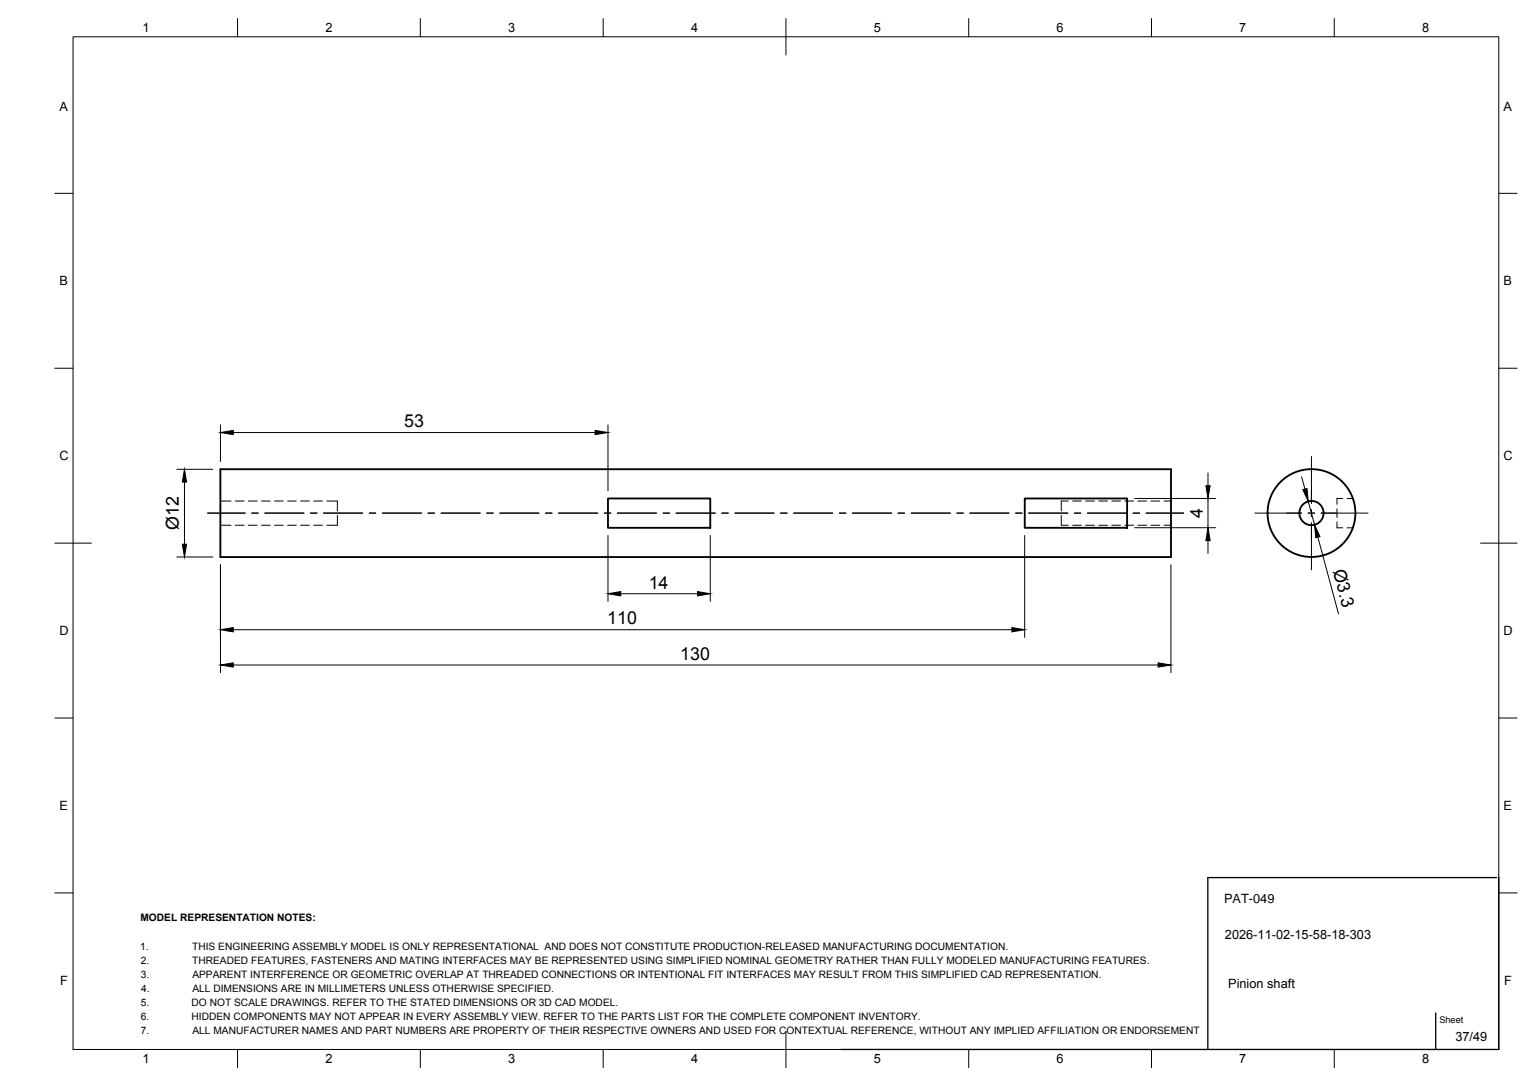
ISO-10303-21;
HEADER;
/* Generated by software containing ST-Developer
 * from STEP Tools, Inc. (www.steptools.com) 
 */

FILE_DESCRIPTION(
/* description */ ('Hand drill press frame (manual)'),
/* implementation_level */ '2;1');

FILE_NAME(
/* name */ 'Pinion shaft.step',
/* time_stamp */ '2026-10-28T03:25:28-07:00',
/* author */ (''),
/* organization */ (''),
/* preprocessor_version */ 'ST-DEVELOPER v20.2',
/* originating_system */ 'Autodesk Translation Framework v15.17.0.0',
/* authorisation */ '');

FILE_SCHEMA (('AUTOMOTIVE_DESIGN { 1 0 10303 214 3 1 1 }'));
ENDSEC;

DATA;
#10=MECHANICAL_DESIGN_GEOMETRIC_PRESENTATION_REPRESENTATION('',(#655),#33299);
#558=SHAPE_REPRESENTATION_RELATIONSHIP('SRR','None',#33520,#603);
#603=ADVANCED_BREP_SHAPE_REPRESENTATION('',(#706),#33282);
#655=STYLED_ITEM('',(#33814),#706);
#706=MANIFOLD_SOLID_BREP('Body1',#12674);
#855=FACE_BOUND('',#2667,.T.);
#856=FACE_BOUND('',#2668,.T.);
#857=FACE_BOUND('',#2670,.T.);
#858=FACE_BOUND('',#2672,.T.);
#1238=PLANE('',#14009);
#1239=PLANE('',#14013);
#1240=PLANE('',#14014);
#1241=PLANE('',#14015);
#1242=PLANE('',#14017);
#1243=PLANE('',#14018);
#1244=PLANE('',#14019);
#1245=PLANE('',#14021);
#1246=PLANE('',#14022);
#1247=PLANE('',#14024);
#1248=PLANE('',#14025);
#1249=PLANE('',#14026);
#1250=PLANE('',#14031);
#1251=PLANE('',#14032);
#1828=FACE_OUTER_BOUND('',#2652,.T.);
#1829=FACE_OUTER_BOUND('',#2653,.T.);
#1830=FACE_OUTER_BOUND('',#2654,.T.);
#1831=FACE_OUTER_BOUND('',#2655,.T.);
#1832=FACE_OUTER_BOUND('',#2656,.T.);
#1833=FACE_OUTER_BOUND('',#2657,.T.);
#1834=FACE_OUTER_BOUND('',#2658,.T.);
#1835=FACE_OUTER_BOUND('',#2659,.T.);
#1836=FACE_OUTER_BOUND('',#2660,.T.);
#1837=FACE_OUTER_BOUND('',#2661,.T.);
#1838=FACE_OUTER_BOUND('',#2662,.T.);
#1839=FACE_OUTER_BOUND('',#2663,.T.);
#1840=FACE_OUTER_BOUND('',#2664,.T.);
#1841=FACE_OUTER_BOUND('',#2665,.T.);
#1842=FACE_OUTER_BOUND('',#2666,.T.);
#1843=FACE_OUTER_BOUND('',#2669,.T.);
#1844=FACE_OUTER_BOUND('',#2671,.T.);
#2652=EDGE_LOOP('',(#10865,#10866,#10867,#10868));
#2653=EDGE_LOOP('',(#10869));
#2654=EDGE_LOOP('',(#10870,#10871,#10872,#10873));
#2655=EDGE_LOOP('',(#10874));
#2656=EDGE_LOOP('',(#10875,#10876,#10877,#10878));
#2657=EDGE_LOOP('',(#10879,#10880,#10881,#10882));
#2658=EDGE_LOOP('',(#10883,#10884,#10885,#10886));
#2659=EDGE_LOOP('',(#10887,#10888,#10889,#10890));
#2660=EDGE_LOOP('',(#10891,#10892,#10893,#10894));
#2661=EDGE_LOOP('',(#10895,#10896,#10897,#10898));
#2662=EDGE_LOOP('',(#10899,#10900,#10901,#10902));
#2663=EDGE_LOOP('',(#10903,#10904,#10905,#10906));
#2664=EDGE_LOOP('',(#10907,#10908,#10909,#10910));
#2665=EDGE_LOOP('',(#10911,#10912,#10913,#10914));
#2666=EDGE_LOOP('',(#10915,#10916,#10917,#10918));
#2667=EDGE_LOOP('',(#10919,#10920,#10921,#10922));
#2668=EDGE_LOOP('',(#10923,#10924,#10925,#10926));
#2669=EDGE_LOOP('',(#10927));
#2670=EDGE_LOOP('',(#10928));
#2671=EDGE_LOOP('',(#10929));
#2672=EDGE_LOOP('',(#10930));
#3785=LINE('',#21071,#4950);
#3786=LINE('',#21078,#4951);
#3787=LINE('',#21084,#4952);
#3788=LINE('',#21086,#4953);
#3789=LINE('',#21088,#4954);
#3790=LINE('',#21089,#4955);
#3791=LINE('',#21094,#4956);
#3792=LINE('',#21095,#4957);
#3793=LINE('',#21098,#4958);
#3794=LINE('',#21099,#4959);
#3795=LINE('',#21102,#4960);
#3796=LINE('',#21103,#4961);
#3797=LINE('',#21109,#4962);
#3798=LINE('',#21111,#4963);
#3799=LINE('',#21113,#4964);
#3800=LINE('',#21114,#4965);
#3801=LINE('',#21119,#4966);
#3802=LINE('',#21120,#4967);
#3803=LINE('',#21123,#4968);
#3804=LINE('',#21124,#4969);
#3805=LINE('',#21127,#4970);
#3806=LINE('',#21128,#4971);
#3807=LINE('',#21135,#4972);
#4950=VECTOR('',#16908,0.165);
#4951=VECTOR('',#16917,0.165);
#4952=VECTOR('',#16924,1.);
#4953=VECTOR('',#16925,1.);
#4954=VECTOR('',#16926,1.);
#4955=VECTOR('',#16927,1.);
#4956=VECTOR('',#16932,1.);
#4957=VECTOR('',#16933,1.);
#4958=VECTOR('',#16936,1.);
#4959=VECTOR('',#16937,1.);
#4960=VECTOR('',#16940,1.);
#4961=VECTOR('',#16941,1.);
#4962=VECTOR('',#16948,1.);
#4963=VECTOR('',#16949,1.);
#4964=VECTOR('',#16950,1.);
#4965=VECTOR('',#16951,1.);
#4966=VECTOR('',#16956,1.);
#4967=VECTOR('',#16957,1.);
#4968=VECTOR('',#16960,1.);
#4969=VECTOR('',#16961,1.);
#4970=VECTOR('',#16964,1.);
#4971=VECTOR('',#16965,1.);
#4972=VECTOR('',#16974,0.6);
#5497=CIRCLE('',#14007,0.165);
#5498=CIRCLE('',#14008,0.165);
#5499=CIRCLE('',#14011,0.165);
#5500=CIRCLE('',#14012,0.165);
#5501=CIRCLE('',#14016,0.6);
#5502=CIRCLE('',#14020,0.6);
#5503=CIRCLE('',#14023,0.6);
#5504=CIRCLE('',#14027,0.6);
#5505=CIRCLE('',#14029,0.6);
#5506=CIRCLE('',#14030,0.6);
#6435=VERTEX_POINT('',#21068);
#6436=VERTEX_POINT('',#21070);
#6437=VERTEX_POINT('',#21075);
#6438=VERTEX_POINT('',#21077);
#6439=VERTEX_POINT('',#21082);
#6440=VERTEX_POINT('',#21083);
#6441=VERTEX_POINT('',#21085);
#6442=VERTEX_POINT('',#21087);
#6443=VERTEX_POINT('',#21091);
#6444=VERTEX_POINT('',#21093);
#6445=VERTEX_POINT('',#21097);
#6446=VERTEX_POINT('',#21101);
#6447=VERTEX_POINT('',#21107);
#6448=VERTEX_POINT('',#21108);
#6449=VERTEX_POINT('',#21110);
#6450=VERTEX_POINT('',#21112);
#6451=VERTEX_POINT('',#21116);
#6452=VERTEX_POINT('',#21118);
#6453=VERTEX_POINT('',#21122);
#6454=VERTEX_POINT('',#21126);
#6455=VERTEX_POINT('',#21132);
#6456=VERTEX_POINT('',#21134);
#7961=EDGE_CURVE('',#6435,#6435,#5497,.T.);
#7962=EDGE_CURVE('',#6435,#6436,#3785,.T.);
#7963=EDGE_CURVE('',#6436,#6436,#5498,.T.);
#7964=EDGE_CURVE('',#6437,#6437,#5499,.T.);
#7965=EDGE_CURVE('',#6437,#6438,#3786,.T.);
#7966=EDGE_CURVE('',#6438,#6438,#5500,.T.);
#7967=EDGE_CURVE('',#6439,#6440,#3787,.T.);
#7968=EDGE_CURVE('',#6439,#6441,#3788,.T.);
#7969=EDGE_CURVE('',#6442,#6441,#3789,.T.);
#7970=EDGE_CURVE('',#6442,#6440,#3790,.T.);
#7971=EDGE_CURVE('',#6440,#6443,#5501,.T.);
#7972=EDGE_CURVE('',#6444,#6442,#3791,.T.);
#7973=EDGE_CURVE('',#6443,#6444,#3792,.T.);
#7974=EDGE_CURVE('',#6441,#6445,#3793,.T.);
#7975=EDGE_CURVE('',#6444,#6445,#3794,.T.);
#7976=EDGE_CURVE('',#6443,#6446,#3795,.T.);
#7977=EDGE_CURVE('',#6445,#6446,#3796,.T.);
#7978=EDGE_CURVE('',#6446,#6439,#5502,.T.);
#7979=EDGE_CURVE('',#6447,#6448,#3797,.T.);
#7980=EDGE_CURVE('',#6447,#6449,#3798,.T.);
#7981=EDGE_CURVE('',#6450,#6449,#3799,.T.);
#7982=EDGE_CURVE('',#6450,#6448,#3800,.T.);
#7983=EDGE_CURVE('',#6448,#6451,#5503,.T.);
#7984=EDGE_CURVE('',#6452,#6450,#3801,.T.);
#7985=EDGE_CURVE('',#6451,#6452,#3802,.T.);
#7986=EDGE_CURVE('',#6449,#6453,#3803,.T.);
#7987=EDGE_CURVE('',#6452,#6453,#3804,.T.);
#7988=EDGE_CURVE('',#6451,#6454,#3805,.T.);
#7989=EDGE_CURVE('',#6453,#6454,#3806,.T.);
#7990=EDGE_CURVE('',#6454,#6447,#5504,.T.);
#7991=EDGE_CURVE('',#6455,#6455,#5505,.T.);
#7992=EDGE_CURVE('',#6455,#6456,#3807,.T.);
#7993=EDGE_CURVE('',#6456,#6456,#5506,.T.);
#10865=ORIENTED_EDGE('',*,*,#7961,.F.);
#10866=ORIENTED_EDGE('',*,*,#7962,.T.);
#10867=ORIENTED_EDGE('',*,*,#7963,.F.);
#10868=ORIENTED_EDGE('',*,*,#7962,.F.);
#10869=ORIENTED_EDGE('',*,*,#7961,.T.);
#10870=ORIENTED_EDGE('',*,*,#7964,.F.);
#10871=ORIENTED_EDGE('',*,*,#7965,.T.);
#10872=ORIENTED_EDGE('',*,*,#7966,.T.);
#10873=ORIENTED_EDGE('',*,*,#7965,.F.);
#10874=ORIENTED_EDGE('',*,*,#7966,.F.);
#10875=ORIENTED_EDGE('',*,*,#7967,.F.);
#10876=ORIENTED_EDGE('',*,*,#7968,.T.);
#10877=ORIENTED_EDGE('',*,*,#7969,.F.);
#10878=ORIENTED_EDGE('',*,*,#7970,.T.);
#10879=ORIENTED_EDGE('',*,*,#7971,.F.);
#10880=ORIENTED_EDGE('',*,*,#7970,.F.);
#10881=ORIENTED_EDGE('',*,*,#7972,.F.);
#10882=ORIENTED_EDGE('',*,*,#7973,.F.);
#10883=ORIENTED_EDGE('',*,*,#7972,.T.);
#10884=ORIENTED_EDGE('',*,*,#7969,.T.);
#10885=ORIENTED_EDGE('',*,*,#7974,.T.);
#10886=ORIENTED_EDGE('',*,*,#7975,.F.);
#10887=ORIENTED_EDGE('',*,*,#7976,.F.);
#10888=ORIENTED_EDGE('',*,*,#7973,.T.);
#10889=ORIENTED_EDGE('',*,*,#7975,.T.);
#10890=ORIENTED_EDGE('',*,*,#7977,.T.);
#10891=ORIENTED_EDGE('',*,*,#7978,.F.);
#10892=ORIENTED_EDGE('',*,*,#7977,.F.);
#10893=ORIENTED_EDGE('',*,*,#7974,.F.);
#10894=ORIENTED_EDGE('',*,*,#7968,.F.);
#10895=ORIENTED_EDGE('',*,*,#7979,.F.);
#10896=ORIENTED_EDGE('',*,*,#7980,.T.);
#10897=ORIENTED_EDGE('',*,*,#7981,.F.);
#10898=ORIENTED_EDGE('',*,*,#7982,.T.);
#10899=ORIENTED_EDGE('',*,*,#7983,.F.);
#10900=ORIENTED_EDGE('',*,*,#7982,.F.);
#10901=ORIENTED_EDGE('',*,*,#7984,.F.);
#10902=ORIENTED_EDGE('',*,*,#7985,.F.);
#10903=ORIENTED_EDGE('',*,*,#7984,.T.);
#10904=ORIENTED_EDGE('',*,*,#7981,.T.);
#10905=ORIENTED_EDGE('',*,*,#7986,.T.);
#10906=ORIENTED_EDGE('',*,*,#7987,.F.);
#10907=ORIENTED_EDGE('',*,*,#7988,.F.);
#10908=ORIENTED_EDGE('',*,*,#7985,.T.);
#10909=ORIENTED_EDGE('',*,*,#7987,.T.);
#10910=ORIENTED_EDGE('',*,*,#7989,.T.);
#10911=ORIENTED_EDGE('',*,*,#7990,.F.);
#10912=ORIENTED_EDGE('',*,*,#7989,.F.);
#10913=ORIENTED_EDGE('',*,*,#7986,.F.);
#10914=ORIENTED_EDGE('',*,*,#7980,.F.);
#10915=ORIENTED_EDGE('',*,*,#7991,.F.);
#10916=ORIENTED_EDGE('',*,*,#7992,.T.);
#10917=ORIENTED_EDGE('',*,*,#7993,.T.);
#10918=ORIENTED_EDGE('',*,*,#7992,.F.);
#10919=ORIENTED_EDGE('',*,*,#7976,.T.);
#10920=ORIENTED_EDGE('',*,*,#7978,.T.);
#10921=ORIENTED_EDGE('',*,*,#7967,.T.);
#10922=ORIENTED_EDGE('',*,*,#7971,.T.);
#10923=ORIENTED_EDGE('',*,*,#7988,.T.);
#10924=ORIENTED_EDGE('',*,*,#7990,.T.);
#10925=ORIENTED_EDGE('',*,*,#7979,.T.);
#10926=ORIENTED_EDGE('',*,*,#7983,.T.);
#10927=ORIENTED_EDGE('',*,*,#7991,.T.);
#10928=ORIENTED_EDGE('',*,*,#7963,.T.);
#10929=ORIENTED_EDGE('',*,*,#7993,.F.);
#10930=ORIENTED_EDGE('',*,*,#7964,.T.);
#11897=CYLINDRICAL_SURFACE('',#14006,0.165);
#11898=CYLINDRICAL_SURFACE('',#14010,0.165);
#11899=CYLINDRICAL_SURFACE('',#14028,0.6);
#12437=ADVANCED_FACE('',(#1828),#11897,.F.);
#12438=ADVANCED_FACE('',(#1829),#1238,.T.);
#12439=ADVANCED_FACE('',(#1830),#11898,.F.);
#12440=ADVANCED_FACE('',(#1831),#1239,.F.);
#12441=ADVANCED_FACE('',(#1832),#1240,.F.);
#12442=ADVANCED_FACE('',(#1833),#1241,.T.);
#12443=ADVANCED_FACE('',(#1834),#1242,.F.);
#12444=ADVANCED_FACE('',(#1835),#1243,.F.);
#12445=ADVANCED_FACE('',(#1836),#1244,.F.);
#12446=ADVANCED_FACE('',(#1837),#1245,.F.);
#12447=ADVANCED_FACE('',(#1838),#1246,.T.);
#12448=ADVANCED_FACE('',(#1839),#1247,.F.);
#12449=ADVANCED_FACE('',(#1840),#1248,.F.);
#12450=ADVANCED_FACE('',(#1841),#1249,.F.);
#12451=ADVANCED_FACE('',(#1842,#855,#856),#11899,.T.);
#12452=ADVANCED_FACE('',(#1843,#857),#1250,.T.);
#12453=ADVANCED_FACE('',(#1844,#858),#1251,.F.);
#12674=CLOSED_SHELL('',(#12437,#12438,#12439,#12440,#12441,#12442,#12443,
#12444,#12445,#12446,#12447,#12448,#12449,#12450,#12451,#12452,#12453));
#14005=AXIS2_PLACEMENT_3D('',#21066,#16902,#16903);
#14006=AXIS2_PLACEMENT_3D('',#21067,#16904,#16905);
#14007=AXIS2_PLACEMENT_3D('',#21069,#16906,#16907);
#14008=AXIS2_PLACEMENT_3D('',#21072,#16909,#16910);
#14009=AXIS2_PLACEMENT_3D('',#21073,#16911,#16912);
#14010=AXIS2_PLACEMENT_3D('',#21074,#16913,#16914);
#14011=AXIS2_PLACEMENT_3D('',#21076,#16915,#16916);
#14012=AXIS2_PLACEMENT_3D('',#21079,#16918,#16919);
#14013=AXIS2_PLACEMENT_3D('',#21080,#16920,#16921);
#14014=AXIS2_PLACEMENT_3D('',#21081,#16922,#16923);
#14015=AXIS2_PLACEMENT_3D('',#21090,#16928,#16929);
#14016=AXIS2_PLACEMENT_3D('',#21092,#16930,#16931);
#14017=AXIS2_PLACEMENT_3D('',#21096,#16934,#16935);
#14018=AXIS2_PLACEMENT_3D('',#21100,#16938,#16939);
#14019=AXIS2_PLACEMENT_3D('',#21104,#16942,#16943);
#14020=AXIS2_PLACEMENT_3D('',#21105,#16944,#16945);
#14021=AXIS2_PLACEMENT_3D('',#21106,#16946,#16947);
#14022=AXIS2_PLACEMENT_3D('',#21115,#16952,#16953);
#14023=AXIS2_PLACEMENT_3D('',#21117,#16954,#16955);
#14024=AXIS2_PLACEMENT_3D('',#21121,#16958,#16959);
#14025=AXIS2_PLACEMENT_3D('',#21125,#16962,#16963);
#14026=AXIS2_PLACEMENT_3D('',#21129,#16966,#16967);
#14027=AXIS2_PLACEMENT_3D('',#21130,#16968,#16969);
#14028=AXIS2_PLACEMENT_3D('',#21131,#16970,#16971);
#14029=AXIS2_PLACEMENT_3D('',#21133,#16972,#16973);
#14030=AXIS2_PLACEMENT_3D('',#21136,#16975,#16976);
#14031=AXIS2_PLACEMENT_3D('',#21137,#16977,#16978);
#14032=AXIS2_PLACEMENT_3D('',#21138,#16979,#16980);
#16902=DIRECTION('axis',(0.,0.,1.));
#16903=DIRECTION('refdir',(1.,0.,0.));
#16904=DIRECTION('center_axis',(0.,1.,0.));
#16905=DIRECTION('ref_axis',(1.,0.,0.));
#16906=DIRECTION('center_axis',(0.,1.,0.));
#16907=DIRECTION('ref_axis',(1.,0.,0.));
#16908=DIRECTION('',(0.,1.,0.));
#16909=DIRECTION('center_axis',(0.,-1.,0.));
#16910=DIRECTION('ref_axis',(1.,0.,0.));
#16911=DIRECTION('center_axis',(0.,1.,0.));
#16912=DIRECTION('ref_axis',(1.,0.,0.));
#16913=DIRECTION('center_axis',(0.,1.,0.));
#16914=DIRECTION('ref_axis',(1.,0.,0.));
#16915=DIRECTION('center_axis',(0.,1.,0.));
#16916=DIRECTION('ref_axis',(1.,0.,0.));
#16917=DIRECTION('',(0.,1.,0.));
#16918=DIRECTION('center_axis',(0.,1.,0.));
#16919=DIRECTION('ref_axis',(1.,0.,0.));
#16920=DIRECTION('center_axis',(0.,1.,0.));
#16921=DIRECTION('ref_axis',(1.,0.,0.));
#16922=DIRECTION('center_axis',(0.,0.,-1.));
#16923=DIRECTION('ref_axis',(-1.,0.,0.));
#16924=DIRECTION('',(0.,-1.,0.));
#16925=DIRECTION('',(-1.,0.,0.));
#16926=DIRECTION('',(0.,1.,0.));
#16927=DIRECTION('',(1.,0.,0.));
#16928=DIRECTION('center_axis',(0.,1.,0.));
#16929=DIRECTION('ref_axis',(1.,0.,0.));
#16930=DIRECTION('center_axis',(0.,-1.,0.));
#16931=DIRECTION('ref_axis',(1.,0.,0.));
#16932=DIRECTION('',(0.,0.,-1.));
#16933=DIRECTION('',(-1.,0.,0.));
#16934=DIRECTION('center_axis',(-1.,0.,0.));
#16935=DIRECTION('ref_axis',(0.,0.,1.));
#16936=DIRECTION('',(0.,0.,1.));
#16937=DIRECTION('',(0.,1.,0.));
#16938=DIRECTION('center_axis',(0.,0.,1.));
#16939=DIRECTION('ref_axis',(1.,0.,0.));
#16940=DIRECTION('',(0.,1.,0.));
#16941=DIRECTION('',(1.,0.,0.));
#16942=DIRECTION('center_axis',(0.,1.,0.));
#16943=DIRECTION('ref_axis',(0.,0.,1.));
#16944=DIRECTION('center_axis',(0.,1.,0.));
#16945=DIRECTION('ref_axis',(1.,0.,0.));
#16946=DIRECTION('center_axis',(0.,0.,-1.));
#16947=DIRECTION('ref_axis',(-1.,0.,0.));
#16948=DIRECTION('',(0.,-1.,0.));
#16949=DIRECTION('',(-1.,0.,0.));
#16950=DIRECTION('',(0.,1.,0.));
#16951=DIRECTION('',(1.,0.,0.));
#16952=DIRECTION('center_axis',(0.,1.,0.));
#16953=DIRECTION('ref_axis',(1.,0.,0.));
#16954=DIRECTION('center_axis',(0.,-1.,0.));
#16955=DIRECTION('ref_axis',(1.,0.,0.));
#16956=DIRECTION('',(0.,0.,-1.));
#16957=DIRECTION('',(-1.,0.,0.));
#16958=DIRECTION('center_axis',(-1.,0.,0.));
#16959=DIRECTION('ref_axis',(0.,0.,1.));
#16960=DIRECTION('',(0.,0.,1.));
#16961=DIRECTION('',(0.,1.,0.));
#16962=DIRECTION('center_axis',(0.,0.,1.));
#16963=DIRECTION('ref_axis',(1.,0.,0.));
#16964=DIRECTION('',(0.,1.,0.));
#16965=DIRECTION('',(1.,0.,0.));
#16966=DIRECTION('center_axis',(0.,1.,0.));
#16967=DIRECTION('ref_axis',(0.,0.,1.));
#16968=DIRECTION('center_axis',(0.,1.,0.));
#16969=DIRECTION('ref_axis',(1.,0.,0.));
#16970=DIRECTION('center_axis',(0.,1.,0.));
#16971=DIRECTION('ref_axis',(1.,0.,0.));
#16972=DIRECTION('center_axis',(0.,1.,0.));
#16973=DIRECTION('ref_axis',(1.,0.,0.));
#16974=DIRECTION('',(0.,-1.,0.));
#16975=DIRECTION('center_axis',(0.,1.,0.));
#16976=DIRECTION('ref_axis',(1.,0.,0.));
#16977=DIRECTION('center_axis',(0.,1.,0.));
#16978=DIRECTION('ref_axis',(1.,0.,0.));
#16979=DIRECTION('center_axis',(0.,1.,0.));
#16980=DIRECTION('ref_axis',(1.,0.,0.));
#21066=CARTESIAN_POINT('',(0.,0.,0.));
#21067=CARTESIAN_POINT('Origin',(-3.25,6.,20.));
#21068=CARTESIAN_POINT('',(-3.415,6.,20.));
#21069=CARTESIAN_POINT('Origin',(-3.25,6.,20.));
#21070=CARTESIAN_POINT('',(-3.415,7.5,20.));
#21071=CARTESIAN_POINT('',(-3.415,6.,20.));
#21072=CARTESIAN_POINT('Origin',(-3.25,7.5,20.));
#21073=CARTESIAN_POINT('Origin',(-3.25,6.,20.));
#21074=CARTESIAN_POINT('Origin',(-3.25,-5.6,20.));
#21075=CARTESIAN_POINT('',(-3.415,-5.5,20.));
#21076=CARTESIAN_POINT('Origin',(-3.25,-5.5,20.));
#21077=CARTESIAN_POINT('',(-3.415,-3.9,20.));
#21078=CARTESIAN_POINT('',(-3.415,-5.6,20.));
#21079=CARTESIAN_POINT('Origin',(-3.25,-3.9,20.));
#21080=CARTESIAN_POINT('Origin',(-3.25,-3.9,20.));
#21081=CARTESIAN_POINT('Origin',(-2.55,5.5,19.8));
#21082=CARTESIAN_POINT('',(-2.68431457505076,6.9,19.8));
#21083=CARTESIAN_POINT('',(-2.68431457505076,5.5,19.8));
#21084=CARTESIAN_POINT('',(-2.68431457505076,-5.5,19.8));
#21085=CARTESIAN_POINT('',(-2.9,6.9,19.8));
#21086=CARTESIAN_POINT('',(-2.9,6.9,19.8));
#21087=CARTESIAN_POINT('',(-2.9,5.5,19.8));
#21088=CARTESIAN_POINT('',(-2.9,5.5,19.8));
#21089=CARTESIAN_POINT('',(-2.9,5.5,19.8));
#21090=CARTESIAN_POINT('Origin',(-2.725,5.5,20.));
#21091=CARTESIAN_POINT('',(-2.68431457505076,5.5,20.2));
#21092=CARTESIAN_POINT('Origin',(-3.25,5.5,20.));
#21093=CARTESIAN_POINT('',(-2.9,5.5,20.2));
#21094=CARTESIAN_POINT('',(-2.9,5.5,20.2));
#21095=CARTESIAN_POINT('',(-2.55,5.5,20.2));
#21096=CARTESIAN_POINT('Origin',(-2.9,5.5,19.8));
#21097=CARTESIAN_POINT('',(-2.9,6.9,20.2));
#21098=CARTESIAN_POINT('',(-2.9,6.9,20.2));
#21099=CARTESIAN_POINT('',(-2.9,5.5,20.2));
#21100=CARTESIAN_POINT('Origin',(-2.9,5.5,20.2));
#21101=CARTESIAN_POINT('',(-2.68431457505076,6.9,20.2));
#21102=CARTESIAN_POINT('',(-2.68431457505076,-5.5,20.2));
#21103=CARTESIAN_POINT('',(-2.55,6.9,20.2));
#21104=CARTESIAN_POINT('Origin',(-2.725,6.9,20.));
#21105=CARTESIAN_POINT('Origin',(-3.25,6.9,20.));
#21106=CARTESIAN_POINT('Origin',(-2.55,-0.2,19.8));
#21107=CARTESIAN_POINT('',(-2.68431457505076,1.2,19.8));
#21108=CARTESIAN_POINT('',(-2.68431457505076,-0.2,19.8));
#21109=CARTESIAN_POINT('',(-2.68431457505076,-5.5,19.8));
#21110=CARTESIAN_POINT('',(-2.9,1.2,19.8));
#21111=CARTESIAN_POINT('',(-2.9,1.2,19.8));
#21112=CARTESIAN_POINT('',(-2.9,-0.2,19.8));
#21113=CARTESIAN_POINT('',(-2.9,-0.2,19.8));
#21114=CARTESIAN_POINT('',(-2.9,-0.2,19.8));
#21115=CARTESIAN_POINT('Origin',(-2.725,-0.2,20.));
#21116=CARTESIAN_POINT('',(-2.68431457505076,-0.2,20.2));
#21117=CARTESIAN_POINT('Origin',(-3.25,-0.2,20.));
#21118=CARTESIAN_POINT('',(-2.9,-0.2,20.2));
#21119=CARTESIAN_POINT('',(-2.9,-0.2,20.2));
#21120=CARTESIAN_POINT('',(-2.55,-0.2,20.2));
#21121=CARTESIAN_POINT('Origin',(-2.9,-0.2,19.8));
#21122=CARTESIAN_POINT('',(-2.9,1.2,20.2));
#21123=CARTESIAN_POINT('',(-2.9,1.2,20.2));
#21124=CARTESIAN_POINT('',(-2.9,-0.2,20.2));
#21125=CARTESIAN_POINT('Origin',(-2.9,-0.2,20.2));
#21126=CARTESIAN_POINT('',(-2.68431457505076,1.2,20.2));
#21127=CARTESIAN_POINT('',(-2.68431457505076,-5.5,20.2));
#21128=CARTESIAN_POINT('',(-2.55,1.2,20.2));
#21129=CARTESIAN_POINT('Origin',(-2.725,1.2,20.));
#21130=CARTESIAN_POINT('Origin',(-3.25,1.2,20.));
#21131=CARTESIAN_POINT('Origin',(-3.25,-5.5,20.));
#21132=CARTESIAN_POINT('',(-3.85,7.5,20.));
#21133=CARTESIAN_POINT('Origin',(-3.25,7.5,20.));
#21134=CARTESIAN_POINT('',(-3.85,-5.5,20.));
#21135=CARTESIAN_POINT('',(-3.85,-5.5,20.));
#21136=CARTESIAN_POINT('Origin',(-3.25,-5.5,20.));
#21137=CARTESIAN_POINT('Origin',(-3.25,7.5,20.));
#21138=CARTESIAN_POINT('Origin',(-3.25,-5.5,20.));
#33230=UNCERTAINTY_MEASURE_WITH_UNIT(LENGTH_MEASURE(0.001),#33300,
'DISTANCE_ACCURACY_VALUE',
'Maximum model space distance between geometric entities at asserted c
onnectivities');
#33247=UNCERTAINTY_MEASURE_WITH_UNIT(LENGTH_MEASURE(0.001),#33300,
'DISTANCE_ACCURACY_VALUE',
'Maximum model space distance between geometric entities at asserted c
onnectivities');
#33282=(
GEOMETRIC_REPRESENTATION_CONTEXT(3)
GLOBAL_UNCERTAINTY_ASSIGNED_CONTEXT((#33230))
GLOBAL_UNIT_ASSIGNED_CONTEXT((#33300,#33302,#33303))
REPRESENTATION_CONTEXT('','3D')
);
#33299=(
GEOMETRIC_REPRESENTATION_CONTEXT(3)
GLOBAL_UNCERTAINTY_ASSIGNED_CONTEXT((#33247))
GLOBAL_UNIT_ASSIGNED_CONTEXT((#33300,#33302,#33303))
REPRESENTATION_CONTEXT('','3D')
);
#33300=(
LENGTH_UNIT()
NAMED_UNIT(*)
SI_UNIT(.CENTI.,.METRE.)
);
#33302=(
NAMED_UNIT(*)
PLANE_ANGLE_UNIT()
SI_UNIT($,.RADIAN.)
);
#33303=(
NAMED_UNIT(*)
SI_UNIT($,.STERADIAN.)
SOLID_ANGLE_UNIT()
);
#33338=SHAPE_DEFINITION_REPRESENTATION(#33400,#33520);
#33400=PRODUCT_DEFINITION_SHAPE('',$,#33572);
#33520=SHAPE_REPRESENTATION('',(#14005),#33282);
#33537=PRODUCT_DEFINITION_CONTEXT('part definition',#33692,'design');
#33572=PRODUCT_DEFINITION('Pinion shaft','Pinion shaft',#33623,#33537);
#33623=PRODUCT_DEFINITION_FORMATION('',$,#33728);
#33692=APPLICATION_CONTEXT(
'Core Data for Automotive Mechanical Design Process');
#33693=PRODUCT_CONTEXT('part definition',#33692,'mechanical');
#33728=PRODUCT('Pinion shaft','Pinion shaft','Pinion shaft',(#33693));
#33808=COLOUR_RGB('Grey',0.48,0.52,0.57);
#33809=FILL_AREA_STYLE_COLOUR('',#33808);
#33810=FILL_AREA_STYLE('',(#33809));
#33811=SURFACE_STYLE_FILL_AREA(#33810);
#33812=SURFACE_SIDE_STYLE('',(#33811));
#33813=SURFACE_STYLE_USAGE(.BOTH.,#33812);
#33814=PRESENTATION_STYLE_ASSIGNMENT((#33813));
ENDSEC;
END-ISO-10303-21;
